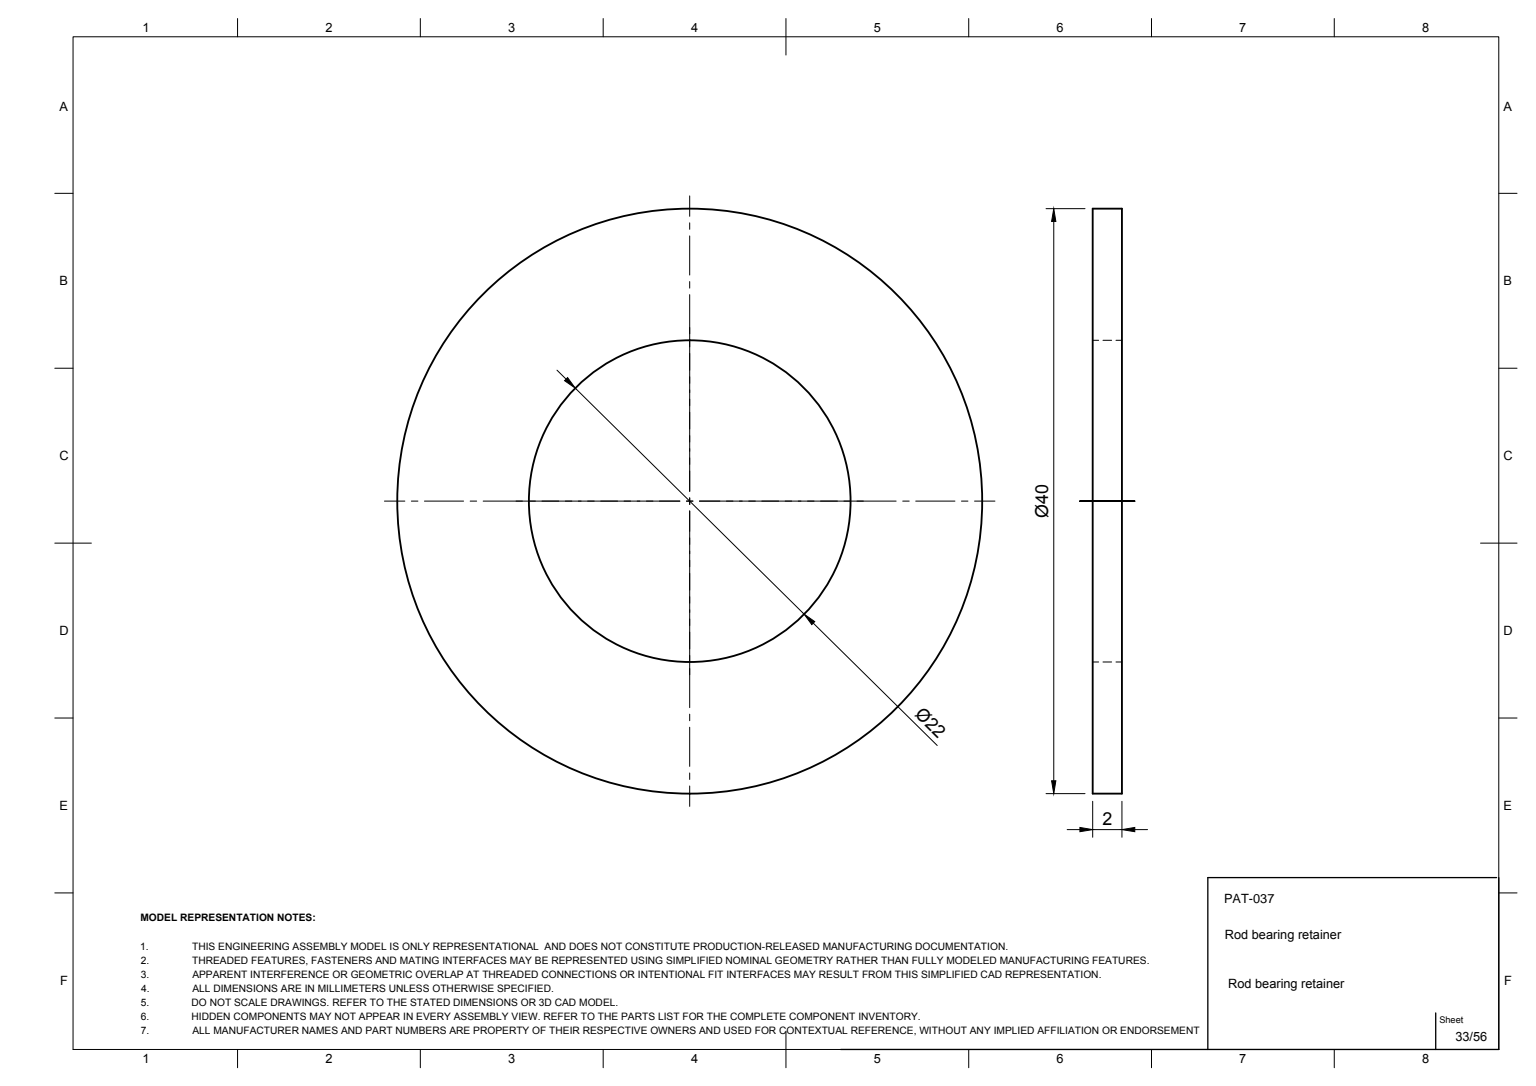
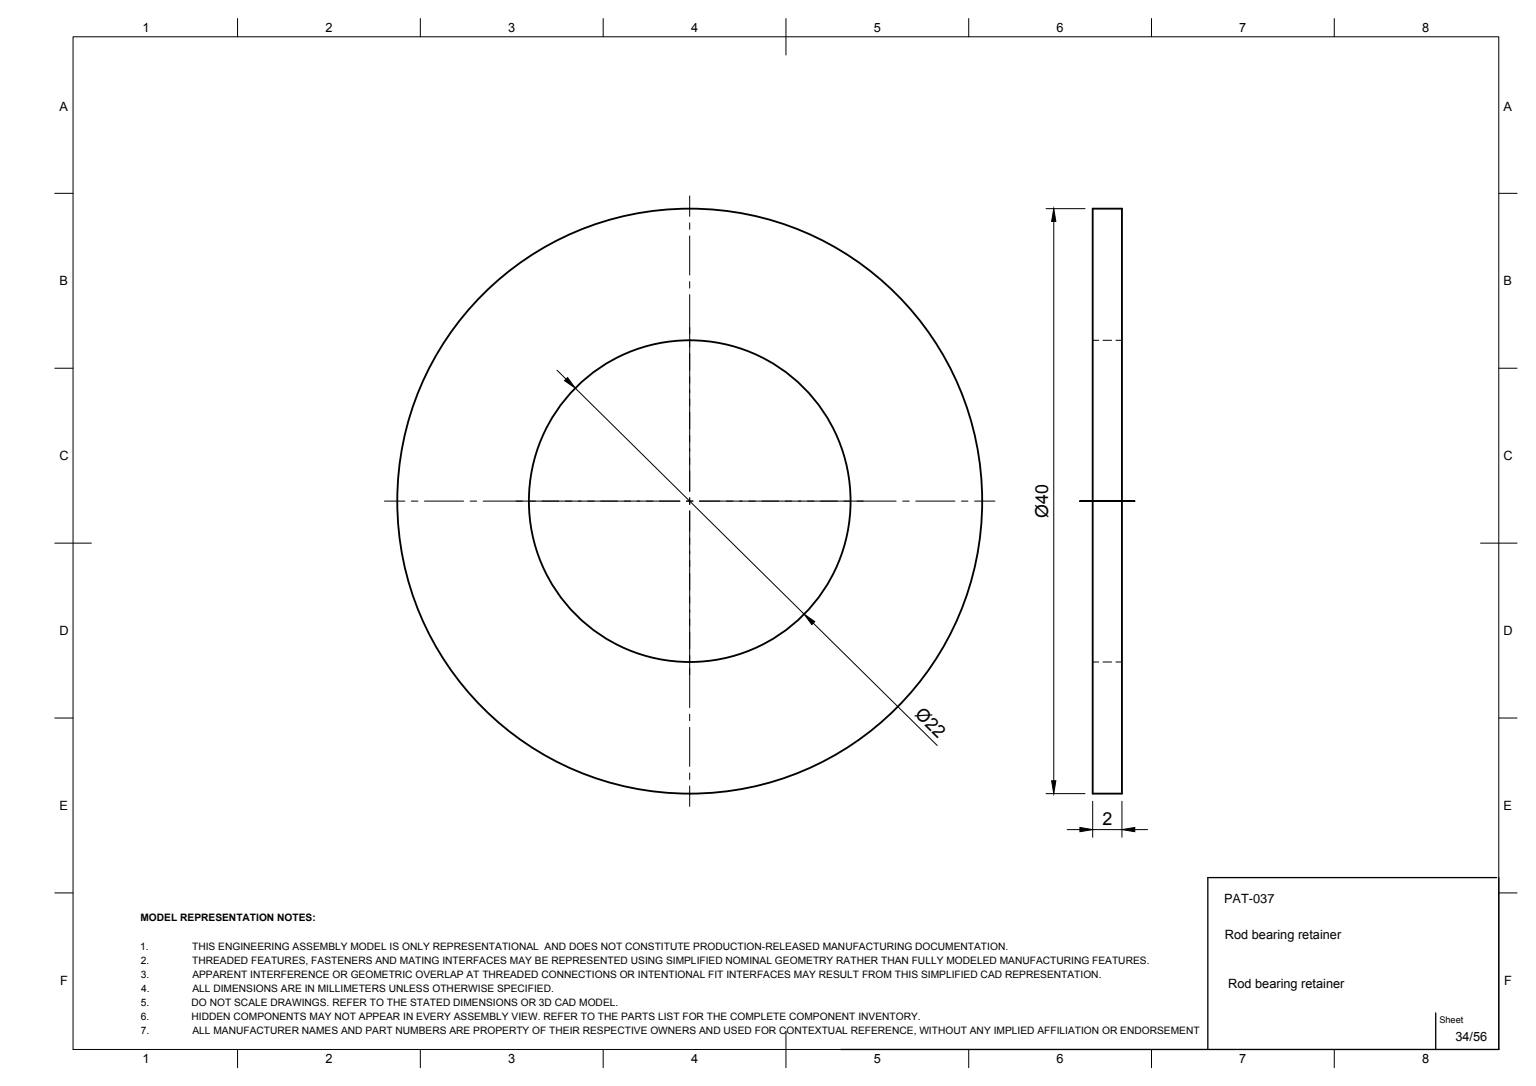
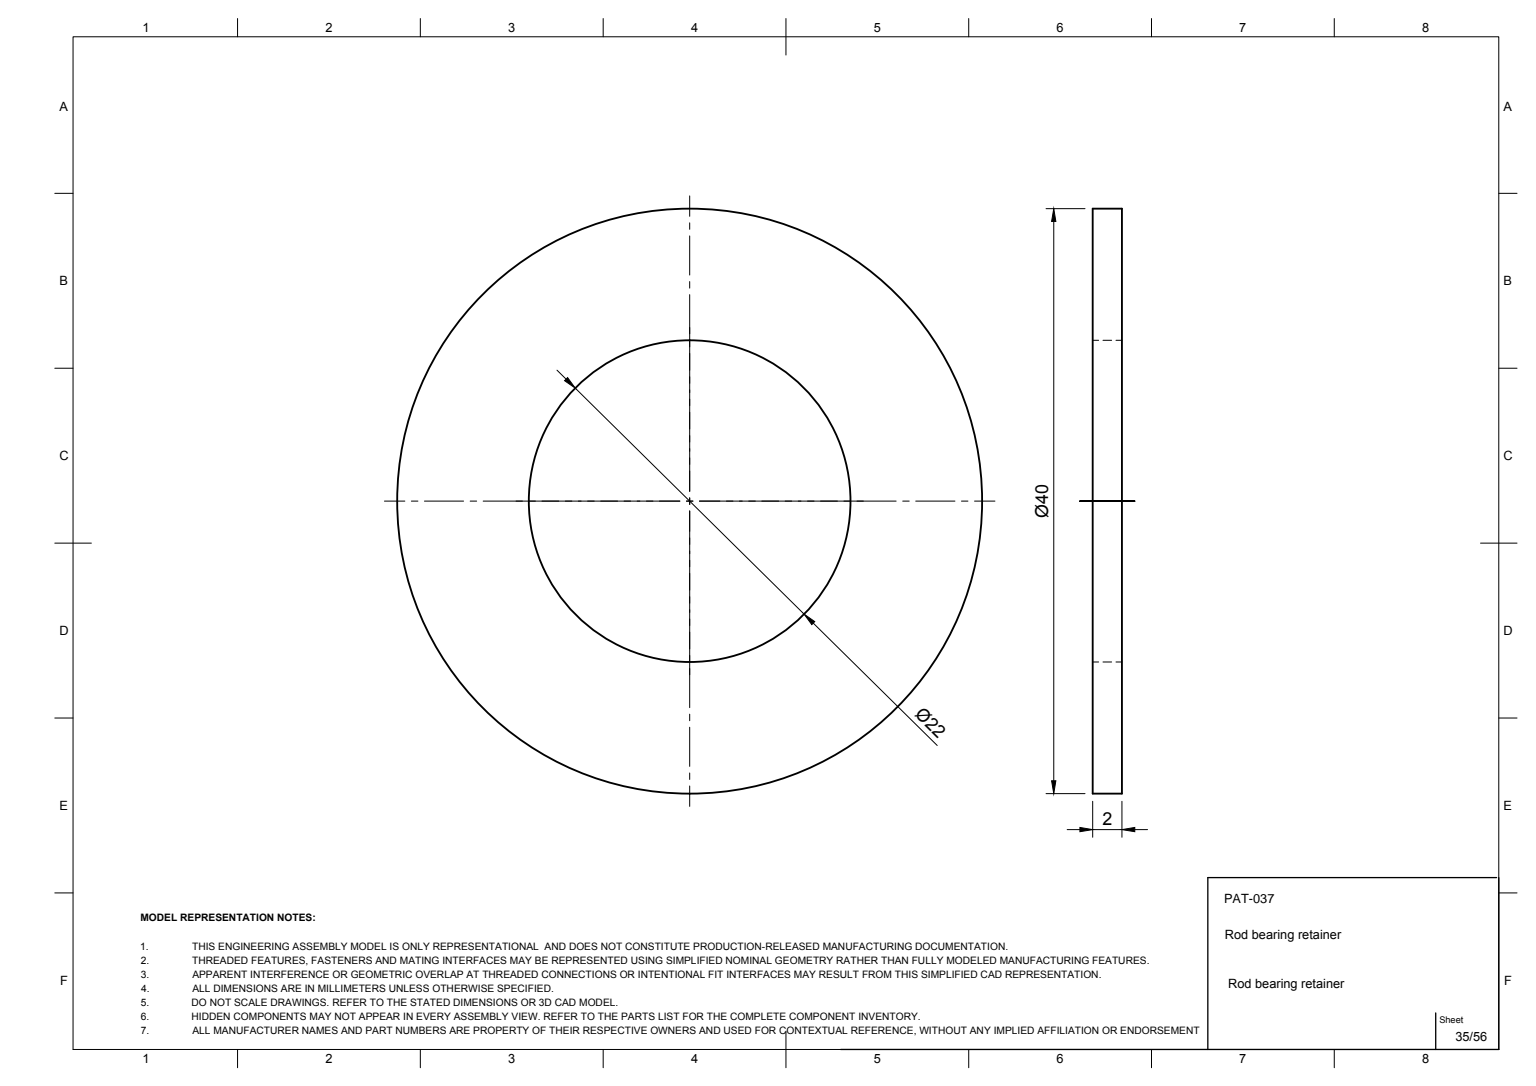
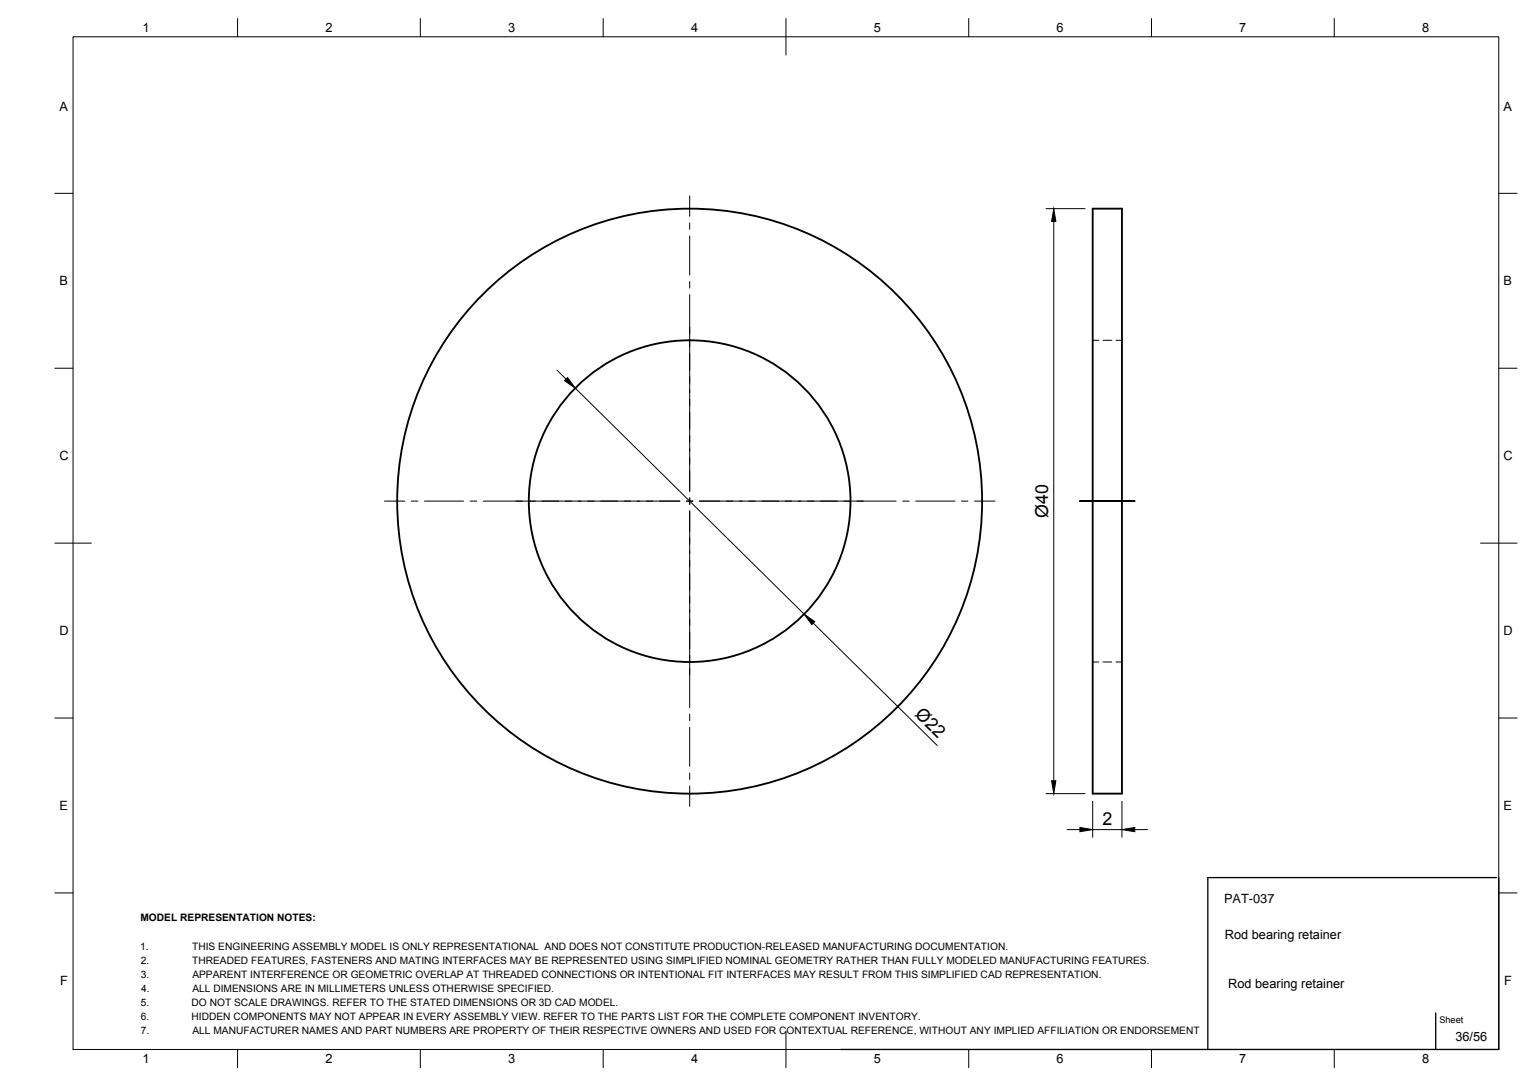
ISO-10303-21;
HEADER;
/* Generated by software containing ST-Developer
 * from STEP Tools, Inc. (www.steptools.com) 
 */

FILE_DESCRIPTION(
/* description */ ('Flywheel Crank-Slider'),
/* implementation_level */ '2;1');

FILE_NAME(
/* name */ 'Rod bearing retainer.step',
/* time_stamp */ '2026-10-28T03:23:13-07:00',
/* author */ (''),
/* organization */ (''),
/* preprocessor_version */ 'ST-DEVELOPER v20.2',
/* originating_system */ 'Autodesk Translation Framework v15.17.0.0',
/* authorisation */ '');

FILE_SCHEMA (('AUTOMOTIVE_DESIGN { 1 0 10303 214 3 1 1 }'));
ENDSEC;

DATA;
#10=MECHANICAL_DESIGN_GEOMETRIC_PRESENTATION_REPRESENTATION('',(#702),#17322);
#597=SHAPE_REPRESENTATION_RELATIONSHIP('SRR','None',#17596,#649);
#649=ADVANCED_BREP_SHAPE_REPRESENTATION('',(#759),#17300);
#702=STYLED_ITEM('',(#17931),#759);
#759=MANIFOLD_SOLID_BREP('Body1',#9084);
#935=FACE_BOUND('',#2374,.T.);
#936=FACE_BOUND('',#2376,.T.);
#1234=PLANE('',#10364);
#1235=PLANE('',#10365);
#1686=FACE_OUTER_BOUND('',#2371,.T.);
#1687=FACE_OUTER_BOUND('',#2372,.T.);
#1688=FACE_OUTER_BOUND('',#2373,.T.);
#1689=FACE_OUTER_BOUND('',#2375,.T.);
#2371=EDGE_LOOP('',(#7650,#7651,#7652,#7653));
#2372=EDGE_LOOP('',(#7654,#7655,#7656,#7657));
#2373=EDGE_LOOP('',(#7658));
#2374=EDGE_LOOP('',(#7659));
#2375=EDGE_LOOP('',(#7660));
#2376=EDGE_LOOP('',(#7661));
#3078=LINE('',#15993,#3689);
#3079=LINE('',#15999,#3690);
#3689=VECTOR('',#12642,1.1);
#3690=VECTOR('',#12649,2.);
#4104=CIRCLE('',#10359,1.1);
#4105=CIRCLE('',#10360,1.1);
#4106=CIRCLE('',#10362,2.);
#4107=CIRCLE('',#10363,2.);
#4783=VERTEX_POINT('',#15990);
#4784=VERTEX_POINT('',#15992);
#4785=VERTEX_POINT('',#15996);
#4786=VERTEX_POINT('',#15998);
#5782=EDGE_CURVE('',#4783,#4783,#4104,.T.);
#5783=EDGE_CURVE('',#4783,#4784,#3078,.T.);
#5784=EDGE_CURVE('',#4784,#4784,#4105,.T.);
#5785=EDGE_CURVE('',#4785,#4785,#4106,.T.);
#5786=EDGE_CURVE('',#4785,#4786,#3079,.T.);
#5787=EDGE_CURVE('',#4786,#4786,#4107,.T.);
#7650=ORIENTED_EDGE('',*,*,#5782,.F.);
#7651=ORIENTED_EDGE('',*,*,#5783,.T.);
#7652=ORIENTED_EDGE('',*,*,#5784,.T.);
#7653=ORIENTED_EDGE('',*,*,#5783,.F.);
#7654=ORIENTED_EDGE('',*,*,#5785,.F.);
#7655=ORIENTED_EDGE('',*,*,#5786,.T.);
#7656=ORIENTED_EDGE('',*,*,#5787,.T.);
#7657=ORIENTED_EDGE('',*,*,#5786,.F.);
#7658=ORIENTED_EDGE('',*,*,#5785,.T.);
#7659=ORIENTED_EDGE('',*,*,#5782,.T.);
#7660=ORIENTED_EDGE('',*,*,#5787,.F.);
#7661=ORIENTED_EDGE('',*,*,#5784,.F.);
#8453=CYLINDRICAL_SURFACE('',#10358,1.1);
#8454=CYLINDRICAL_SURFACE('',#10361,2.);
#8877=ADVANCED_FACE('',(#1686),#8453,.F.);
#8878=ADVANCED_FACE('',(#1687),#8454,.T.);
#8879=ADVANCED_FACE('',(#1688,#935),#1234,.T.);
#8880=ADVANCED_FACE('',(#1689,#936),#1235,.F.);
#9084=CLOSED_SHELL('',(#8877,#8878,#8879,#8880));
#10357=AXIS2_PLACEMENT_3D('',#15988,#12636,#12637);
#10358=AXIS2_PLACEMENT_3D('',#15989,#12638,#12639);
#10359=AXIS2_PLACEMENT_3D('',#15991,#12640,#12641);
#10360=AXIS2_PLACEMENT_3D('',#15994,#12643,#12644);
#10361=AXIS2_PLACEMENT_3D('',#15995,#12645,#12646);
#10362=AXIS2_PLACEMENT_3D('',#15997,#12647,#12648);
#10363=AXIS2_PLACEMENT_3D('',#16000,#12650,#12651);
#10364=AXIS2_PLACEMENT_3D('',#16001,#12652,#12653);
#10365=AXIS2_PLACEMENT_3D('',#16002,#12654,#12655);
#12636=DIRECTION('axis',(0.,0.,1.));
#12637=DIRECTION('refdir',(1.,0.,0.));
#12638=DIRECTION('center_axis',(0.,1.,0.));
#12639=DIRECTION('ref_axis',(1.,0.,0.));
#12640=DIRECTION('center_axis',(0.,-1.,0.));
#12641=DIRECTION('ref_axis',(1.,0.,0.));
#12642=DIRECTION('',(0.,-1.,0.));
#12643=DIRECTION('center_axis',(0.,-1.,0.));
#12644=DIRECTION('ref_axis',(1.,0.,0.));
#12645=DIRECTION('center_axis',(0.,1.,0.));
#12646=DIRECTION('ref_axis',(1.,0.,0.));
#12647=DIRECTION('center_axis',(0.,1.,0.));
#12648=DIRECTION('ref_axis',(1.,0.,0.));
#12649=DIRECTION('',(0.,-1.,0.));
#12650=DIRECTION('center_axis',(0.,1.,0.));
#12651=DIRECTION('ref_axis',(1.,0.,0.));
#12652=DIRECTION('center_axis',(0.,1.,0.));
#12653=DIRECTION('ref_axis',(1.,0.,0.));
#12654=DIRECTION('center_axis',(0.,1.,0.));
#12655=DIRECTION('ref_axis',(1.,0.,0.));
#15988=CARTESIAN_POINT('',(0.,0.,0.));
#15989=CARTESIAN_POINT('Origin',(2.,2.3,10.));
#15990=CARTESIAN_POINT('',(0.9,2.5,10.));
#15991=CARTESIAN_POINT('Origin',(2.,2.5,10.));
#15992=CARTESIAN_POINT('',(0.9,2.3,10.));
#15993=CARTESIAN_POINT('',(0.9,2.3,10.));
#15994=CARTESIAN_POINT('Origin',(2.,2.3,10.));
#15995=CARTESIAN_POINT('Origin',(2.,2.3,10.));
#15996=CARTESIAN_POINT('',(0.,2.5,10.));
#15997=CARTESIAN_POINT('Origin',(2.,2.5,10.));
#15998=CARTESIAN_POINT('',(0.,2.3,10.));
#15999=CARTESIAN_POINT('',(0.,2.3,10.));
#16000=CARTESIAN_POINT('Origin',(2.,2.3,10.));
#16001=CARTESIAN_POINT('Origin',(2.,2.5,10.));
#16002=CARTESIAN_POINT('Origin',(2.,2.3,10.));
#17239=UNCERTAINTY_MEASURE_WITH_UNIT(LENGTH_MEASURE(0.001),#17323,
'DISTANCE_ACCURACY_VALUE',
'Maximum model space distance between geometric entities at asserted c
onnectivities');
#17261=UNCERTAINTY_MEASURE_WITH_UNIT(LENGTH_MEASURE(0.001),#17323,
'DISTANCE_ACCURACY_VALUE',
'Maximum model space distance between geometric entities at asserted c
onnectivities');
#17300=(
GEOMETRIC_REPRESENTATION_CONTEXT(3)
GLOBAL_UNCERTAINTY_ASSIGNED_CONTEXT((#17239))
GLOBAL_UNIT_ASSIGNED_CONTEXT((#17323,#17325,#17326))
REPRESENTATION_CONTEXT('','3D')
);
#17322=(
GEOMETRIC_REPRESENTATION_CONTEXT(3)
GLOBAL_UNCERTAINTY_ASSIGNED_CONTEXT((#17261))
GLOBAL_UNIT_ASSIGNED_CONTEXT((#17323,#17325,#17326))
REPRESENTATION_CONTEXT('','3D')
);
#17323=(
LENGTH_UNIT()
NAMED_UNIT(*)
SI_UNIT(.CENTI.,.METRE.)
);
#17325=(
NAMED_UNIT(*)
PLANE_ANGLE_UNIT()
SI_UNIT($,.RADIAN.)
);
#17326=(
NAMED_UNIT(*)
SI_UNIT($,.STERADIAN.)
SOLID_ANGLE_UNIT()
);
#17365=SHAPE_DEFINITION_REPRESENTATION(#17427,#17596);
#17427=PRODUCT_DEFINITION_SHAPE('',$,#17657);
#17596=SHAPE_REPRESENTATION('',(#10357),#17300);
#17618=PRODUCT_DEFINITION_CONTEXT('part definition',#17800,'design');
#17657=PRODUCT_DEFINITION('Rod bearing retainer','Rod bearing retainer',
#17717,#17618);
#17717=PRODUCT_DEFINITION_FORMATION('',$,#17840);
#17800=APPLICATION_CONTEXT(
'Core Data for Automotive Mechanical Design Process');
#17801=PRODUCT_CONTEXT('part definition',#17800,'mechanical');
#17840=PRODUCT('Rod bearing retainer','Rod bearing retainer',
'Rod bearing retainer',(#17801));
#17925=COLOUR_RGB('Grey',0.48,0.52,0.57);
#17926=FILL_AREA_STYLE_COLOUR('',#17925);
#17927=FILL_AREA_STYLE('',(#17926));
#17928=SURFACE_STYLE_FILL_AREA(#17927);
#17929=SURFACE_SIDE_STYLE('',(#17928));
#17930=SURFACE_STYLE_USAGE(.BOTH.,#17929);
#17931=PRESENTATION_STYLE_ASSIGNMENT((#17930));
ENDSEC;
END-ISO-10303-21;
